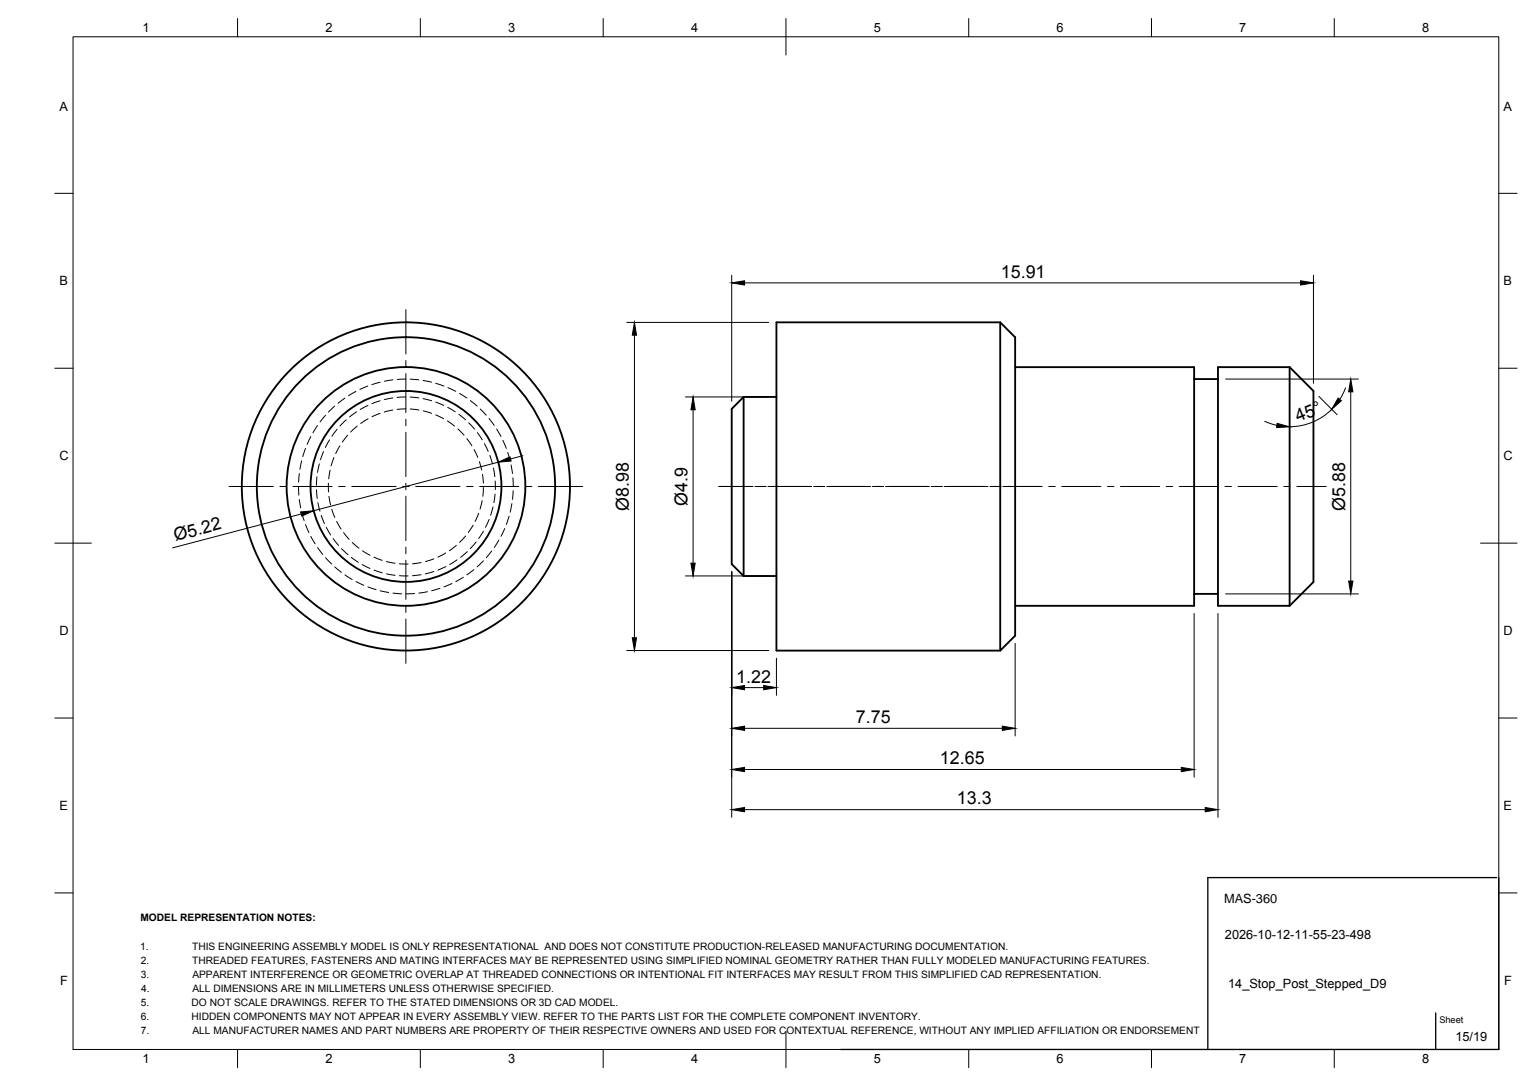
ISO-10303-21;
HEADER;
/* Generated by software containing ST-Developer
 * from STEP Tools, Inc. (www.steptools.com) 
 */

FILE_DESCRIPTION(
/* description */ (''),
/* implementation_level */ '2;1');

FILE_NAME(
/* name */ '14_Stop_Post_Stepped_D9.step',
/* time_stamp */ '2026-11-04T18:53:29-08:00',
/* author */ (''),
/* organization */ (''),
/* preprocessor_version */ 'ST-DEVELOPER v20.2',
/* originating_system */ 'Autodesk Translation Framework v15.17.0.0',
/* authorisation */ '');

FILE_SCHEMA (('AUTOMOTIVE_DESIGN { 1 0 10303 214 3 1 1 }'));
ENDSEC;

DATA;
#10=MECHANICAL_DESIGN_GEOMETRIC_PRESENTATION_REPRESENTATION('',(#1341),#100031);
#243=CONICAL_SURFACE('',#22440,2.2848,0.785398163397448);
#244=CONICAL_SURFACE('',#22448,4.284,0.785398163397447);
#245=CONICAL_SURFACE('',#22462,2.9376,0.785398163397446);
#1156=CIRCLE('',#22439,2.1216);
#1157=CIRCLE('',#22441,2.448);
#1158=CIRCLE('',#22443,2.448);
#1159=CIRCLE('',#22445,4.488);
#1160=CIRCLE('',#22447,4.488);
#1161=CIRCLE('',#22449,4.08);
#1162=CIRCLE('',#22451,3.264);
#1163=CIRCLE('',#22453,3.264);
#1164=CIRCLE('',#22455,2.9376);
#1165=CIRCLE('',#22457,2.9376);
#1166=CIRCLE('',#22459,3.264);
#1167=CIRCLE('',#22461,3.264);
#1168=CIRCLE('',#22463,2.6112);
#1305=SHAPE_REPRESENTATION_RELATIONSHIP('SRR','None',#100115,#1323);
#1323=ADVANCED_BREP_SHAPE_REPRESENTATION('',(#1359),#100027);
#1341=STYLED_ITEM('',(#100200),#1359);
#1359=MANIFOLD_SOLID_BREP('Body1',#20131);
#1681=PLANE('',#22438);
#1682=PLANE('',#22444);
#1683=PLANE('',#22450);
#1684=PLANE('',#22454);
#1685=PLANE('',#22458);
#1686=PLANE('',#22464);
#1804=FACE_BOUND('',#7423,.T.);
#1805=FACE_BOUND('',#7427,.T.);
#1806=FACE_BOUND('',#7430,.T.);
#1807=FACE_BOUND('',#7433,.T.);
#3251=LINE('',#99868,#4538);
#3252=LINE('',#99872,#4539);
#3253=LINE('',#99879,#4540);
#3254=LINE('',#99882,#4541);
#3255=LINE('',#99890,#4542);
#3256=LINE('',#99897,#4543);
#3257=LINE('',#99904,#4544);
#3258=LINE('',#99907,#4545);
#4538=VECTOR('',#28012,2.2848);
#4539=VECTOR('',#28017,2.448);
#4540=VECTOR('',#28026,4.488);
#4541=VECTOR('',#28029,4.284);
#4542=VECTOR('',#28040,3.264);
#4543=VECTOR('',#28049,2.9376);
#4544=VECTOR('',#28058,3.264);
#4545=VECTOR('',#28061,2.9376);
#5017=CYLINDRICAL_SURFACE('',#22442,2.448);
#5018=CYLINDRICAL_SURFACE('',#22446,4.488);
#5019=CYLINDRICAL_SURFACE('',#22452,3.264);
#5020=CYLINDRICAL_SURFACE('',#22456,2.9376);
#5021=CYLINDRICAL_SURFACE('',#22460,3.264);
#6152=FACE_OUTER_BOUND('',#7419,.T.);
#6153=FACE_OUTER_BOUND('',#7420,.T.);
#6154=FACE_OUTER_BOUND('',#7421,.T.);
#6155=FACE_OUTER_BOUND('',#7422,.T.);
#6156=FACE_OUTER_BOUND('',#7424,.T.);
#6157=FACE_OUTER_BOUND('',#7425,.T.);
#6158=FACE_OUTER_BOUND('',#7426,.T.);
#6159=FACE_OUTER_BOUND('',#7428,.T.);
#6160=FACE_OUTER_BOUND('',#7429,.T.);
#6161=FACE_OUTER_BOUND('',#7431,.T.);
#6162=FACE_OUTER_BOUND('',#7432,.T.);
#6163=FACE_OUTER_BOUND('',#7434,.T.);
#6164=FACE_OUTER_BOUND('',#7435,.T.);
#6165=FACE_OUTER_BOUND('',#7436,.T.);
#7419=EDGE_LOOP('',(#18763));
#7420=EDGE_LOOP('',(#18764,#18765,#18766,#18767));
#7421=EDGE_LOOP('',(#18768,#18769,#18770,#18771));
#7422=EDGE_LOOP('',(#18772));
#7423=EDGE_LOOP('',(#18773));
#7424=EDGE_LOOP('',(#18774,#18775,#18776,#18777));
#7425=EDGE_LOOP('',(#18778,#18779,#18780,#18781));
#7426=EDGE_LOOP('',(#18782));
#7427=EDGE_LOOP('',(#18783));
#7428=EDGE_LOOP('',(#18784,#18785,#18786,#18787));
#7429=EDGE_LOOP('',(#18788));
#7430=EDGE_LOOP('',(#18789));
#7431=EDGE_LOOP('',(#18790,#18791,#18792,#18793));
#7432=EDGE_LOOP('',(#18794));
#7433=EDGE_LOOP('',(#18795));
#7434=EDGE_LOOP('',(#18796,#18797,#18798,#18799));
#7435=EDGE_LOOP('',(#18800,#18801,#18802,#18803));
#7436=EDGE_LOOP('',(#18804));
#9897=VERTEX_POINT('',#99863);
#9898=VERTEX_POINT('',#99866);
#9899=VERTEX_POINT('',#99870);
#9900=VERTEX_POINT('',#99874);
#9901=VERTEX_POINT('',#99877);
#9902=VERTEX_POINT('',#99881);
#9903=VERTEX_POINT('',#99885);
#9904=VERTEX_POINT('',#99888);
#9905=VERTEX_POINT('',#99892);
#9906=VERTEX_POINT('',#99895);
#9907=VERTEX_POINT('',#99899);
#9908=VERTEX_POINT('',#99902);
#9909=VERTEX_POINT('',#99906);
#12856=EDGE_CURVE('',#9897,#9897,#1156,.T.);
#12857=EDGE_CURVE('',#9898,#9898,#1157,.T.);
#12858=EDGE_CURVE('',#9898,#9897,#3251,.T.);
#12859=EDGE_CURVE('',#9899,#9899,#1158,.T.);
#12860=EDGE_CURVE('',#9899,#9898,#3252,.T.);
#12861=EDGE_CURVE('',#9900,#9900,#1159,.T.);
#12862=EDGE_CURVE('',#9901,#9901,#1160,.T.);
#12863=EDGE_CURVE('',#9901,#9900,#3253,.T.);
#12864=EDGE_CURVE('',#9901,#9902,#3254,.T.);
#12865=EDGE_CURVE('',#9902,#9902,#1161,.T.);
#12866=EDGE_CURVE('',#9903,#9903,#1162,.T.);
#12867=EDGE_CURVE('',#9904,#9904,#1163,.T.);
#12868=EDGE_CURVE('',#9904,#9903,#3255,.T.);
#12869=EDGE_CURVE('',#9905,#9905,#1164,.T.);
#12870=EDGE_CURVE('',#9906,#9906,#1165,.T.);
#12871=EDGE_CURVE('',#9906,#9905,#3256,.T.);
#12872=EDGE_CURVE('',#9907,#9907,#1166,.T.);
#12873=EDGE_CURVE('',#9908,#9908,#1167,.T.);
#12874=EDGE_CURVE('',#9908,#9907,#3257,.T.);
#12875=EDGE_CURVE('',#9908,#9909,#3258,.T.);
#12876=EDGE_CURVE('',#9909,#9909,#1168,.T.);
#18763=ORIENTED_EDGE('',*,*,#12856,.F.);
#18764=ORIENTED_EDGE('',*,*,#12857,.F.);
#18765=ORIENTED_EDGE('',*,*,#12858,.T.);
#18766=ORIENTED_EDGE('',*,*,#12856,.T.);
#18767=ORIENTED_EDGE('',*,*,#12858,.F.);
#18768=ORIENTED_EDGE('',*,*,#12859,.F.);
#18769=ORIENTED_EDGE('',*,*,#12860,.T.);
#18770=ORIENTED_EDGE('',*,*,#12857,.T.);
#18771=ORIENTED_EDGE('',*,*,#12860,.F.);
#18772=ORIENTED_EDGE('',*,*,#12861,.F.);
#18773=ORIENTED_EDGE('',*,*,#12859,.T.);
#18774=ORIENTED_EDGE('',*,*,#12862,.F.);
#18775=ORIENTED_EDGE('',*,*,#12863,.T.);
#18776=ORIENTED_EDGE('',*,*,#12861,.T.);
#18777=ORIENTED_EDGE('',*,*,#12863,.F.);
#18778=ORIENTED_EDGE('',*,*,#12862,.T.);
#18779=ORIENTED_EDGE('',*,*,#12864,.T.);
#18780=ORIENTED_EDGE('',*,*,#12865,.F.);
#18781=ORIENTED_EDGE('',*,*,#12864,.F.);
#18782=ORIENTED_EDGE('',*,*,#12865,.T.);
#18783=ORIENTED_EDGE('',*,*,#12866,.F.);
#18784=ORIENTED_EDGE('',*,*,#12867,.F.);
#18785=ORIENTED_EDGE('',*,*,#12868,.T.);
#18786=ORIENTED_EDGE('',*,*,#12866,.T.);
#18787=ORIENTED_EDGE('',*,*,#12868,.F.);
#18788=ORIENTED_EDGE('',*,*,#12867,.T.);
#18789=ORIENTED_EDGE('',*,*,#12869,.F.);
#18790=ORIENTED_EDGE('',*,*,#12870,.F.);
#18791=ORIENTED_EDGE('',*,*,#12871,.T.);
#18792=ORIENTED_EDGE('',*,*,#12869,.T.);
#18793=ORIENTED_EDGE('',*,*,#12871,.F.);
#18794=ORIENTED_EDGE('',*,*,#12872,.F.);
#18795=ORIENTED_EDGE('',*,*,#12870,.T.);
#18796=ORIENTED_EDGE('',*,*,#12873,.F.);
#18797=ORIENTED_EDGE('',*,*,#12874,.T.);
#18798=ORIENTED_EDGE('',*,*,#12872,.T.);
#18799=ORIENTED_EDGE('',*,*,#12874,.F.);
#18800=ORIENTED_EDGE('',*,*,#12873,.T.);
#18801=ORIENTED_EDGE('',*,*,#12875,.T.);
#18802=ORIENTED_EDGE('',*,*,#12876,.F.);
#18803=ORIENTED_EDGE('',*,*,#12875,.F.);
#18804=ORIENTED_EDGE('',*,*,#12876,.T.);
#20086=ADVANCED_FACE('',(#6152),#1681,.T.);
#20087=ADVANCED_FACE('',(#6153),#243,.T.);
#20088=ADVANCED_FACE('',(#6154),#5017,.T.);
#20089=ADVANCED_FACE('',(#6155,#1804),#1682,.T.);
#20090=ADVANCED_FACE('',(#6156),#5018,.T.);
#20091=ADVANCED_FACE('',(#6157),#244,.T.);
#20092=ADVANCED_FACE('',(#6158,#1805),#1683,.T.);
#20093=ADVANCED_FACE('',(#6159),#5019,.T.);
#20094=ADVANCED_FACE('',(#6160,#1806),#1684,.T.);
#20095=ADVANCED_FACE('',(#6161),#5020,.T.);
#20096=ADVANCED_FACE('',(#6162,#1807),#1685,.T.);
#20097=ADVANCED_FACE('',(#6163),#5021,.T.);
#20098=ADVANCED_FACE('',(#6164),#245,.T.);
#20099=ADVANCED_FACE('',(#6165),#1686,.T.);
#20131=CLOSED_SHELL('',(#20086,#20087,#20088,#20089,#20090,#20091,#20092,
#20093,#20094,#20095,#20096,#20097,#20098,#20099));
#22437=AXIS2_PLACEMENT_3D('',#99861,#28002,#28003);
#22438=AXIS2_PLACEMENT_3D('',#99862,#28004,#28005);
#22439=AXIS2_PLACEMENT_3D('',#99864,#28006,#28007);
#22440=AXIS2_PLACEMENT_3D('',#99865,#28008,#28009);
#22441=AXIS2_PLACEMENT_3D('',#99867,#28010,#28011);
#22442=AXIS2_PLACEMENT_3D('',#99869,#28013,#28014);
#22443=AXIS2_PLACEMENT_3D('',#99871,#28015,#28016);
#22444=AXIS2_PLACEMENT_3D('',#99873,#28018,#28019);
#22445=AXIS2_PLACEMENT_3D('',#99875,#28020,#28021);
#22446=AXIS2_PLACEMENT_3D('',#99876,#28022,#28023);
#22447=AXIS2_PLACEMENT_3D('',#99878,#28024,#28025);
#22448=AXIS2_PLACEMENT_3D('',#99880,#28027,#28028);
#22449=AXIS2_PLACEMENT_3D('',#99883,#28030,#28031);
#22450=AXIS2_PLACEMENT_3D('',#99884,#28032,#28033);
#22451=AXIS2_PLACEMENT_3D('',#99886,#28034,#28035);
#22452=AXIS2_PLACEMENT_3D('',#99887,#28036,#28037);
#22453=AXIS2_PLACEMENT_3D('',#99889,#28038,#28039);
#22454=AXIS2_PLACEMENT_3D('',#99891,#28041,#28042);
#22455=AXIS2_PLACEMENT_3D('',#99893,#28043,#28044);
#22456=AXIS2_PLACEMENT_3D('',#99894,#28045,#28046);
#22457=AXIS2_PLACEMENT_3D('',#99896,#28047,#28048);
#22458=AXIS2_PLACEMENT_3D('',#99898,#28050,#28051);
#22459=AXIS2_PLACEMENT_3D('',#99900,#28052,#28053);
#22460=AXIS2_PLACEMENT_3D('',#99901,#28054,#28055);
#22461=AXIS2_PLACEMENT_3D('',#99903,#28056,#28057);
#22462=AXIS2_PLACEMENT_3D('',#99905,#28059,#28060);
#22463=AXIS2_PLACEMENT_3D('',#99908,#28062,#28063);
#22464=AXIS2_PLACEMENT_3D('',#99909,#28064,#28065);
#28002=DIRECTION('axis',(0.,0.,1.));
#28003=DIRECTION('refdir',(1.,0.,0.));
#28004=DIRECTION('center_axis',(-1.,0.,0.));
#28005=DIRECTION('ref_axis',(0.,0.,1.));
#28006=DIRECTION('center_axis',(1.,0.,0.));
#28007=DIRECTION('ref_axis',(0.,0.,-1.));
#28008=DIRECTION('center_axis',(1.,0.,0.));
#28009=DIRECTION('ref_axis',(0.,1.,0.));
#28010=DIRECTION('center_axis',(1.,0.,0.));
#28011=DIRECTION('ref_axis',(0.,0.,-1.));
#28012=DIRECTION('',(-0.707106781186548,0.707106781186547,8.65956056235493E-17));
#28013=DIRECTION('center_axis',(1.,0.,0.));
#28014=DIRECTION('ref_axis',(0.,1.,0.));
#28015=DIRECTION('center_axis',(1.,0.,0.));
#28016=DIRECTION('ref_axis',(0.,0.,-1.));
#28017=DIRECTION('',(-1.,0.,0.));
#28018=DIRECTION('center_axis',(-1.,0.,0.));
#28019=DIRECTION('ref_axis',(0.,0.,1.));
#28020=DIRECTION('center_axis',(1.,0.,0.));
#28021=DIRECTION('ref_axis',(0.,0.,-1.));
#28022=DIRECTION('center_axis',(1.,0.,0.));
#28023=DIRECTION('ref_axis',(0.,1.,0.));
#28024=DIRECTION('center_axis',(1.,0.,0.));
#28025=DIRECTION('ref_axis',(0.,0.,-1.));
#28026=DIRECTION('',(-1.,0.,0.));
#28027=DIRECTION('center_axis',(-1.,0.,0.));
#28028=DIRECTION('ref_axis',(0.,1.,0.));
#28029=DIRECTION('',(0.707106781186548,0.707106781186547,-8.65956056235492E-17));
#28030=DIRECTION('center_axis',(1.,0.,0.));
#28031=DIRECTION('ref_axis',(0.,0.,-1.));
#28032=DIRECTION('center_axis',(1.,0.,0.));
#28033=DIRECTION('ref_axis',(0.,0.,-1.));
#28034=DIRECTION('center_axis',(1.,0.,0.));
#28035=DIRECTION('ref_axis',(0.,0.,-1.));
#28036=DIRECTION('center_axis',(1.,0.,0.));
#28037=DIRECTION('ref_axis',(0.,1.,0.));
#28038=DIRECTION('center_axis',(1.,0.,0.));
#28039=DIRECTION('ref_axis',(0.,0.,-1.));
#28040=DIRECTION('',(-1.,0.,0.));
#28041=DIRECTION('center_axis',(1.,0.,0.));
#28042=DIRECTION('ref_axis',(0.,0.,-1.));
#28043=DIRECTION('center_axis',(1.,0.,0.));
#28044=DIRECTION('ref_axis',(0.,0.,-1.));
#28045=DIRECTION('center_axis',(1.,0.,0.));
#28046=DIRECTION('ref_axis',(0.,1.,0.));
#28047=DIRECTION('center_axis',(1.,0.,0.));
#28048=DIRECTION('ref_axis',(0.,0.,-1.));
#28049=DIRECTION('',(-1.,0.,0.));
#28050=DIRECTION('center_axis',(-1.,0.,0.));
#28051=DIRECTION('ref_axis',(0.,0.,1.));
#28052=DIRECTION('center_axis',(1.,0.,0.));
#28053=DIRECTION('ref_axis',(0.,0.,-1.));
#28054=DIRECTION('center_axis',(1.,0.,0.));
#28055=DIRECTION('ref_axis',(0.,1.,0.));
#28056=DIRECTION('center_axis',(1.,0.,0.));
#28057=DIRECTION('ref_axis',(0.,0.,-1.));
#28058=DIRECTION('',(-1.,0.,0.));
#28059=DIRECTION('center_axis',(-1.,0.,0.));
#28060=DIRECTION('ref_axis',(0.,1.,0.));
#28061=DIRECTION('',(0.707106781186549,0.707106781186546,-8.65956056235491E-17));
#28062=DIRECTION('center_axis',(1.,0.,0.));
#28063=DIRECTION('ref_axis',(0.,0.,-1.));
#28064=DIRECTION('center_axis',(1.,0.,0.));
#28065=DIRECTION('ref_axis',(0.,0.,-1.));
#99861=CARTESIAN_POINT('',(0.,0.,0.));
#99862=CARTESIAN_POINT('Origin',(0.,2.1216,0.));
#99863=CARTESIAN_POINT('',(5.20417042793042E-16,-2.1216,-2.59821064907102E-16));
#99864=CARTESIAN_POINT('Origin',(0.,0.,0.));
#99865=CARTESIAN_POINT('Origin',(0.163200000000001,0.,0.));
#99866=CARTESIAN_POINT('',(0.326400000000001,-2.448,-2.99793536431272E-16));
#99867=CARTESIAN_POINT('Origin',(0.3264,0.,0.));
#99868=CARTESIAN_POINT('',(0.163200000000001,-2.2848,-2.79807300669187E-16));
#99869=CARTESIAN_POINT('Origin',(0.7752,0.,0.));
#99870=CARTESIAN_POINT('',(1.224,-2.448,-2.99793536431272E-16));
#99871=CARTESIAN_POINT('Origin',(1.224,0.,0.));
#99872=CARTESIAN_POINT('',(0.7752,-2.448,-2.99793536431272E-16));
#99873=CARTESIAN_POINT('Origin',(1.224,4.488,0.));
#99874=CARTESIAN_POINT('',(1.224,-4.488,-5.49621483457332E-16));
#99875=CARTESIAN_POINT('Origin',(1.224,0.,0.));
#99876=CARTESIAN_POINT('Origin',(4.284,0.,0.));
#99877=CARTESIAN_POINT('',(7.344,-4.488,-5.49621483457332E-16));
#99878=CARTESIAN_POINT('Origin',(7.344,0.,0.));
#99879=CARTESIAN_POINT('',(4.284,-4.488,-5.49621483457332E-16));
#99880=CARTESIAN_POINT('Origin',(7.548,0.,0.));
#99881=CARTESIAN_POINT('',(7.752,-4.08,-4.9965589405212E-16));
#99882=CARTESIAN_POINT('',(7.548,-4.284,5.24638688754726E-16));
#99883=CARTESIAN_POINT('Origin',(7.752,0.,0.));
#99884=CARTESIAN_POINT('Origin',(7.752,3.264,0.));
#99885=CARTESIAN_POINT('',(7.752,-3.264,-3.99724715241696E-16));
#99886=CARTESIAN_POINT('Origin',(7.752,0.,0.));
#99887=CARTESIAN_POINT('Origin',(10.2,0.,0.));
#99888=CARTESIAN_POINT('',(12.648,-3.264,-3.99724715241696E-16));
#99889=CARTESIAN_POINT('Origin',(12.648,0.,0.));
#99890=CARTESIAN_POINT('',(10.2,-3.264,-3.99724715241696E-16));
#99891=CARTESIAN_POINT('Origin',(12.648,2.9376,0.));
#99892=CARTESIAN_POINT('',(12.648,-2.9376,-3.59752243717526E-16));
#99893=CARTESIAN_POINT('Origin',(12.648,0.,0.));
#99894=CARTESIAN_POINT('Origin',(12.9744,0.,0.));
#99895=CARTESIAN_POINT('',(13.3008,-2.9376,-3.59752243717526E-16));
#99896=CARTESIAN_POINT('Origin',(13.3008,0.,0.));
#99897=CARTESIAN_POINT('',(12.9744,-2.9376,-3.59752243717527E-16));
#99898=CARTESIAN_POINT('Origin',(13.3008,3.264,0.));
#99899=CARTESIAN_POINT('',(13.3008,-3.264,-3.99724715241696E-16));
#99900=CARTESIAN_POINT('Origin',(13.3008,0.,0.));
#99901=CARTESIAN_POINT('Origin',(14.28,0.,0.));
#99902=CARTESIAN_POINT('',(15.2592,-3.264,-3.99724715241696E-16));
#99903=CARTESIAN_POINT('Origin',(15.2592,0.,0.));
#99904=CARTESIAN_POINT('',(14.28,-3.264,-3.99724715241696E-16));
#99905=CARTESIAN_POINT('Origin',(15.5856,0.,0.));
#99906=CARTESIAN_POINT('',(15.912,-2.6112,-3.19779772193357E-16));
#99907=CARTESIAN_POINT('',(15.5856,-2.9376,3.59752243717527E-16));
#99908=CARTESIAN_POINT('Origin',(15.912,0.,0.));
#99909=CARTESIAN_POINT('Origin',(15.912,0.,0.));
#100007=UNCERTAINTY_MEASURE_WITH_UNIT(LENGTH_MEASURE(0.01),#100032,
'DISTANCE_ACCURACY_VALUE',
'Maximum model space distance between geometric entities at asserted c
onnectivities');
#100011=UNCERTAINTY_MEASURE_WITH_UNIT(LENGTH_MEASURE(0.01),#100032,
'DISTANCE_ACCURACY_VALUE',
'Maximum model space distance between geometric entities at asserted c
onnectivities');
#100027=(
GEOMETRIC_REPRESENTATION_CONTEXT(3)
GLOBAL_UNCERTAINTY_ASSIGNED_CONTEXT((#100007))
GLOBAL_UNIT_ASSIGNED_CONTEXT((#100032,#100034,#100035))
REPRESENTATION_CONTEXT('','3D')
);
#100031=(
GEOMETRIC_REPRESENTATION_CONTEXT(3)
GLOBAL_UNCERTAINTY_ASSIGNED_CONTEXT((#100011))
GLOBAL_UNIT_ASSIGNED_CONTEXT((#100032,#100034,#100035))
REPRESENTATION_CONTEXT('','3D')
);
#100032=(
LENGTH_UNIT()
NAMED_UNIT(*)
SI_UNIT(.MILLI.,.METRE.)
);
#100034=(
NAMED_UNIT(*)
PLANE_ANGLE_UNIT()
SI_UNIT($,.RADIAN.)
);
#100035=(
NAMED_UNIT(*)
SI_UNIT($,.STERADIAN.)
SOLID_ANGLE_UNIT()
);
#100051=SHAPE_DEFINITION_REPRESENTATION(#100070,#100115);
#100070=PRODUCT_DEFINITION_SHAPE('',$,#100135);
#100115=SHAPE_REPRESENTATION('',(#22437),#100027);
#100119=PRODUCT_DEFINITION_CONTEXT('part definition',#100178,'design');
#100135=PRODUCT_DEFINITION('2026-10-12-11-55-23-498',
'14_Stop_Post_Stepped_D9',#100154,#100119);
#100154=PRODUCT_DEFINITION_FORMATION('',$,#100195);
#100178=APPLICATION_CONTEXT(
'Core Data for Automotive Mechanical Design Process');
#100179=PRODUCT_CONTEXT('part definition',#100178,'mechanical');
#100195=PRODUCT('2026-10-12-11-55-23-498','14_Stop_Post_Stepped_D9',$,(#100179));
#100200=PRESENTATION_STYLE_ASSIGNMENT((#100206));
#100206=SURFACE_STYLE_USAGE(.BOTH.,#100212);
#100212=SURFACE_SIDE_STYLE('',(#100218));
#100218=SURFACE_STYLE_FILL_AREA(#100224);
#100224=FILL_AREA_STYLE('Opaque(227,224,212)',(#100230));
#100230=FILL_AREA_STYLE_COLOUR('Opaque(227,224,212)',#100236);
#100236=COLOUR_RGB('Opaque(227,224,212)',0.890196078431372,0.87843137254902,
0.831372549019608);
ENDSEC;
END-ISO-10303-21;
